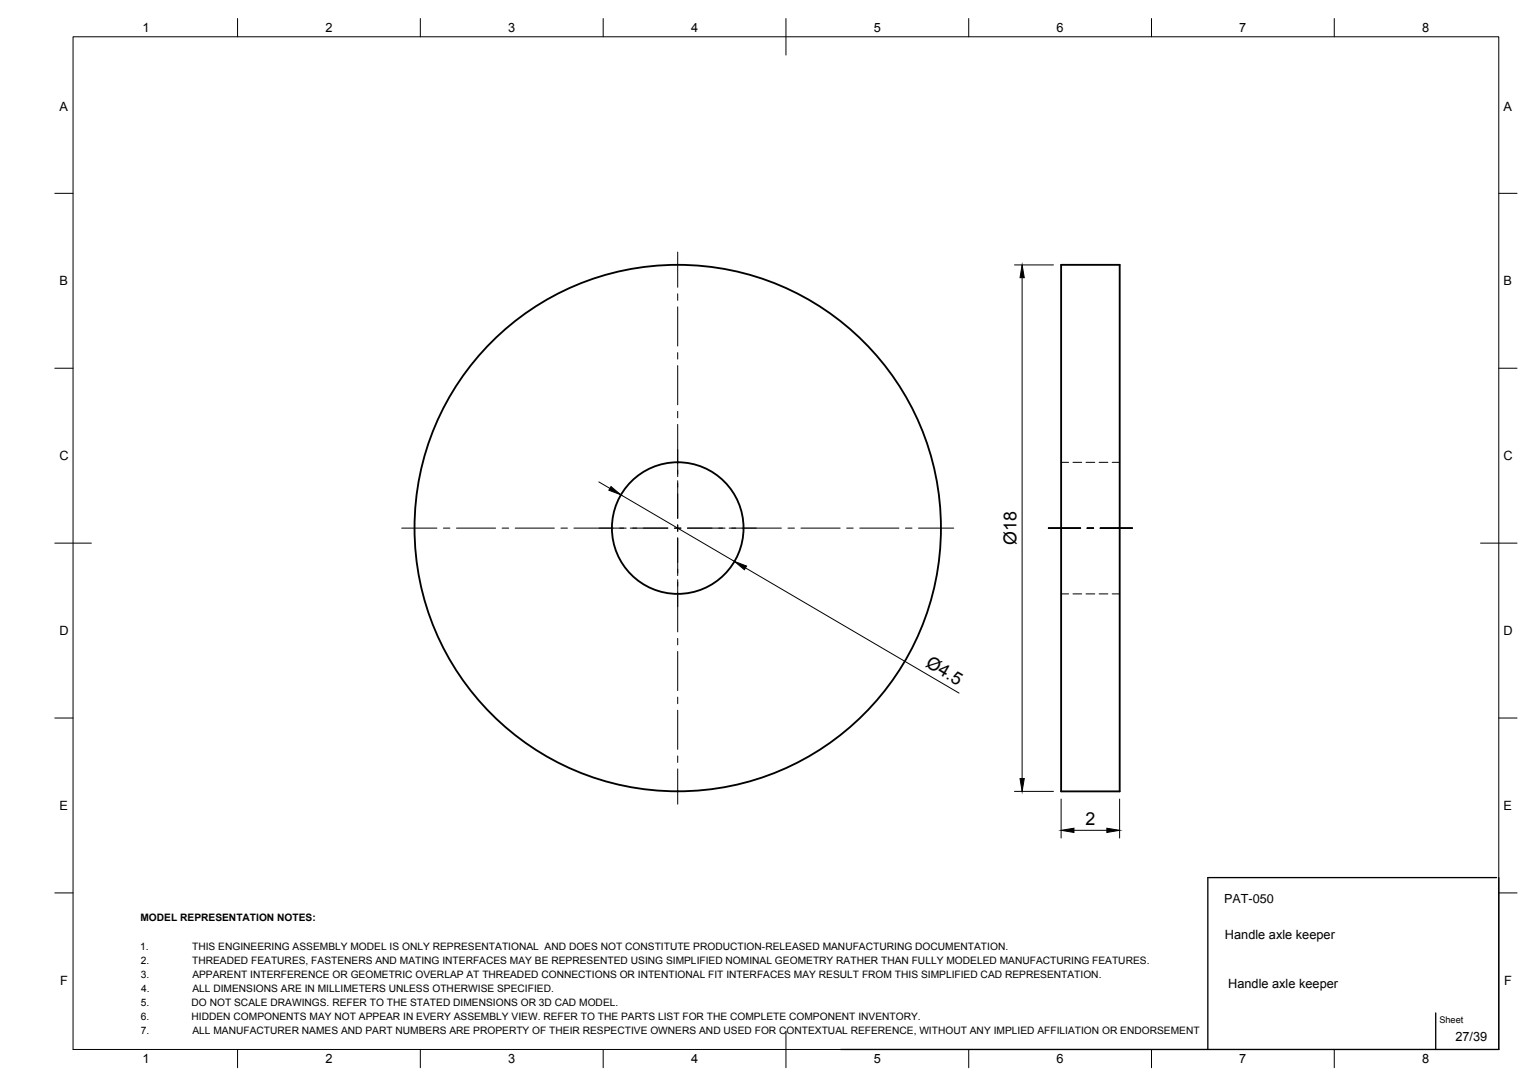
ISO-10303-21;
HEADER;
/* Generated by software containing ST-Developer
 * from STEP Tools, Inc. (www.steptools.com) 
 */

FILE_DESCRIPTION(
/* description */ ('Hand wheel with handle and shaft collar'),
/* implementation_level */ '2;1');

FILE_NAME(
/* name */ 'Handle axle keeper.step',
/* time_stamp */ '2026-10-28T03:23:19-07:00',
/* author */ (''),
/* organization */ (''),
/* preprocessor_version */ 'ST-DEVELOPER v20.2',
/* originating_system */ 'Autodesk Translation Framework v15.17.0.0',
/* authorisation */ '');

FILE_SCHEMA (('AUTOMOTIVE_DESIGN { 1 0 10303 214 3 1 1 }'));
ENDSEC;

DATA;
#10=MECHANICAL_DESIGN_GEOMETRIC_PRESENTATION_REPRESENTATION('',(#422),#10510);
#351=SHAPE_REPRESENTATION_RELATIONSHIP('SRR','None',#10669,#383);
#383=ADVANCED_BREP_SHAPE_REPRESENTATION('',(#468),#10496);
#422=STYLED_ITEM('',(#10908),#468);
#468=MANIFOLD_SOLID_BREP('Body1',#5322);
#579=FACE_BOUND('',#1373,.T.);
#580=FACE_BOUND('',#1375,.T.);
#700=PLANE('',#6126);
#701=PLANE('',#6127);
#958=FACE_OUTER_BOUND('',#1370,.T.);
#959=FACE_OUTER_BOUND('',#1371,.T.);
#960=FACE_OUTER_BOUND('',#1372,.T.);
#961=FACE_OUTER_BOUND('',#1374,.T.);
#1370=EDGE_LOOP('',(#4395,#4396,#4397,#4398));
#1371=EDGE_LOOP('',(#4399,#4400,#4401,#4402));
#1372=EDGE_LOOP('',(#4403));
#1373=EDGE_LOOP('',(#4404));
#1374=EDGE_LOOP('',(#4405));
#1375=EDGE_LOOP('',(#4406));
#1712=LINE('',#9506,#2022);
#1713=LINE('',#9512,#2023);
#2022=VECTOR('',#7468,0.225);
#2023=VECTOR('',#7475,0.9);
#2331=CIRCLE('',#6121,0.225);
#2332=CIRCLE('',#6122,0.225);
#2333=CIRCLE('',#6124,0.9);
#2334=CIRCLE('',#6125,0.9);
#2731=VERTEX_POINT('',#9503);
#2732=VERTEX_POINT('',#9505);
#2733=VERTEX_POINT('',#9509);
#2734=VERTEX_POINT('',#9511);
#3315=EDGE_CURVE('',#2731,#2731,#2331,.T.);
#3316=EDGE_CURVE('',#2731,#2732,#1712,.T.);
#3317=EDGE_CURVE('',#2732,#2732,#2332,.T.);
#3318=EDGE_CURVE('',#2733,#2733,#2333,.T.);
#3319=EDGE_CURVE('',#2733,#2734,#1713,.T.);
#3320=EDGE_CURVE('',#2734,#2734,#2334,.T.);
#4395=ORIENTED_EDGE('',*,*,#3315,.F.);
#4396=ORIENTED_EDGE('',*,*,#3316,.T.);
#4397=ORIENTED_EDGE('',*,*,#3317,.T.);
#4398=ORIENTED_EDGE('',*,*,#3316,.F.);
#4399=ORIENTED_EDGE('',*,*,#3318,.F.);
#4400=ORIENTED_EDGE('',*,*,#3319,.T.);
#4401=ORIENTED_EDGE('',*,*,#3320,.T.);
#4402=ORIENTED_EDGE('',*,*,#3319,.F.);
#4403=ORIENTED_EDGE('',*,*,#3318,.T.);
#4404=ORIENTED_EDGE('',*,*,#3315,.T.);
#4405=ORIENTED_EDGE('',*,*,#3320,.F.);
#4406=ORIENTED_EDGE('',*,*,#3317,.F.);
#4949=CYLINDRICAL_SURFACE('',#6120,0.225);
#4950=CYLINDRICAL_SURFACE('',#6123,0.9);
#5170=ADVANCED_FACE('',(#958),#4949,.F.);
#5171=ADVANCED_FACE('',(#959),#4950,.T.);
#5172=ADVANCED_FACE('',(#960,#579),#700,.T.);
#5173=ADVANCED_FACE('',(#961,#580),#701,.F.);
#5322=CLOSED_SHELL('',(#5170,#5171,#5172,#5173));
#6119=AXIS2_PLACEMENT_3D('',#9501,#7462,#7463);
#6120=AXIS2_PLACEMENT_3D('',#9502,#7464,#7465);
#6121=AXIS2_PLACEMENT_3D('',#9504,#7466,#7467);
#6122=AXIS2_PLACEMENT_3D('',#9507,#7469,#7470);
#6123=AXIS2_PLACEMENT_3D('',#9508,#7471,#7472);
#6124=AXIS2_PLACEMENT_3D('',#9510,#7473,#7474);
#6125=AXIS2_PLACEMENT_3D('',#9513,#7476,#7477);
#6126=AXIS2_PLACEMENT_3D('',#9514,#7478,#7479);
#6127=AXIS2_PLACEMENT_3D('',#9515,#7480,#7481);
#7462=DIRECTION('axis',(0.,0.,1.));
#7463=DIRECTION('refdir',(1.,0.,0.));
#7464=DIRECTION('center_axis',(0.,1.,0.));
#7465=DIRECTION('ref_axis',(1.,0.,0.));
#7466=DIRECTION('center_axis',(0.,-1.,0.));
#7467=DIRECTION('ref_axis',(1.,0.,0.));
#7468=DIRECTION('',(0.,-1.,0.));
#7469=DIRECTION('center_axis',(0.,-1.,0.));
#7470=DIRECTION('ref_axis',(1.,0.,0.));
#7471=DIRECTION('center_axis',(0.,1.,0.));
#7472=DIRECTION('ref_axis',(1.,0.,0.));
#7473=DIRECTION('center_axis',(0.,1.,0.));
#7474=DIRECTION('ref_axis',(1.,0.,0.));
#7475=DIRECTION('',(0.,-1.,0.));
#7476=DIRECTION('center_axis',(0.,1.,0.));
#7477=DIRECTION('ref_axis',(1.,0.,0.));
#7478=DIRECTION('center_axis',(0.,1.,0.));
#7479=DIRECTION('ref_axis',(1.,0.,0.));
#7480=DIRECTION('center_axis',(0.,1.,0.));
#7481=DIRECTION('ref_axis',(1.,0.,0.));
#9501=CARTESIAN_POINT('',(0.,0.,0.));
#9502=CARTESIAN_POINT('Origin',(6.5,-6.2,10.));
#9503=CARTESIAN_POINT('',(6.275,-6.,10.));
#9504=CARTESIAN_POINT('Origin',(6.5,-6.,10.));
#9505=CARTESIAN_POINT('',(6.275,-6.2,10.));
#9506=CARTESIAN_POINT('',(6.275,-6.2,10.));
#9507=CARTESIAN_POINT('Origin',(6.5,-6.2,10.));
#9508=CARTESIAN_POINT('Origin',(6.5,-6.2,10.));
#9509=CARTESIAN_POINT('',(5.6,-6.,10.));
#9510=CARTESIAN_POINT('Origin',(6.5,-6.,10.));
#9511=CARTESIAN_POINT('',(5.6,-6.2,10.));
#9512=CARTESIAN_POINT('',(5.6,-6.2,10.));
#9513=CARTESIAN_POINT('Origin',(6.5,-6.2,10.));
#9514=CARTESIAN_POINT('Origin',(6.5,-6.,10.));
#9515=CARTESIAN_POINT('Origin',(6.5,-6.2,10.));
#10457=UNCERTAINTY_MEASURE_WITH_UNIT(LENGTH_MEASURE(0.001),#10511,
'DISTANCE_ACCURACY_VALUE',
'Maximum model space distance between geometric entities at asserted c
onnectivities');
#10471=UNCERTAINTY_MEASURE_WITH_UNIT(LENGTH_MEASURE(0.001),#10511,
'DISTANCE_ACCURACY_VALUE',
'Maximum model space distance between geometric entities at asserted c
onnectivities');
#10496=(
GEOMETRIC_REPRESENTATION_CONTEXT(3)
GLOBAL_UNCERTAINTY_ASSIGNED_CONTEXT((#10457))
GLOBAL_UNIT_ASSIGNED_CONTEXT((#10511,#10513,#10514))
REPRESENTATION_CONTEXT('','3D')
);
#10510=(
GEOMETRIC_REPRESENTATION_CONTEXT(3)
GLOBAL_UNCERTAINTY_ASSIGNED_CONTEXT((#10471))
GLOBAL_UNIT_ASSIGNED_CONTEXT((#10511,#10513,#10514))
REPRESENTATION_CONTEXT('','3D')
);
#10511=(
LENGTH_UNIT()
NAMED_UNIT(*)
SI_UNIT(.CENTI.,.METRE.)
);
#10513=(
NAMED_UNIT(*)
PLANE_ANGLE_UNIT()
SI_UNIT($,.RADIAN.)
);
#10514=(
NAMED_UNIT(*)
SI_UNIT($,.STERADIAN.)
SOLID_ANGLE_UNIT()
);
#10539=SHAPE_DEFINITION_REPRESENTATION(#10582,#10669);
#10582=PRODUCT_DEFINITION_SHAPE('',$,#10708);
#10669=SHAPE_REPRESENTATION('',(#6119),#10496);
#10683=PRODUCT_DEFINITION_CONTEXT('part definition',#10799,'design');
#10708=PRODUCT_DEFINITION('Handle axle keeper','Handle axle keeper',#10746,
#10683);
#10746=PRODUCT_DEFINITION_FORMATION('',$,#10825);
#10799=APPLICATION_CONTEXT(
'Core Data for Automotive Mechanical Design Process');
#10800=PRODUCT_CONTEXT('part definition',#10799,'mechanical');
#10825=PRODUCT('Handle axle keeper','Handle axle keeper',
'Handle axle keeper',(#10800));
#10902=COLOUR_RGB('Grey',0.48,0.52,0.57);
#10903=FILL_AREA_STYLE_COLOUR('',#10902);
#10904=FILL_AREA_STYLE('',(#10903));
#10905=SURFACE_STYLE_FILL_AREA(#10904);
#10906=SURFACE_SIDE_STYLE('',(#10905));
#10907=SURFACE_STYLE_USAGE(.BOTH.,#10906);
#10908=PRESENTATION_STYLE_ASSIGNMENT((#10907));
ENDSEC;
END-ISO-10303-21;
